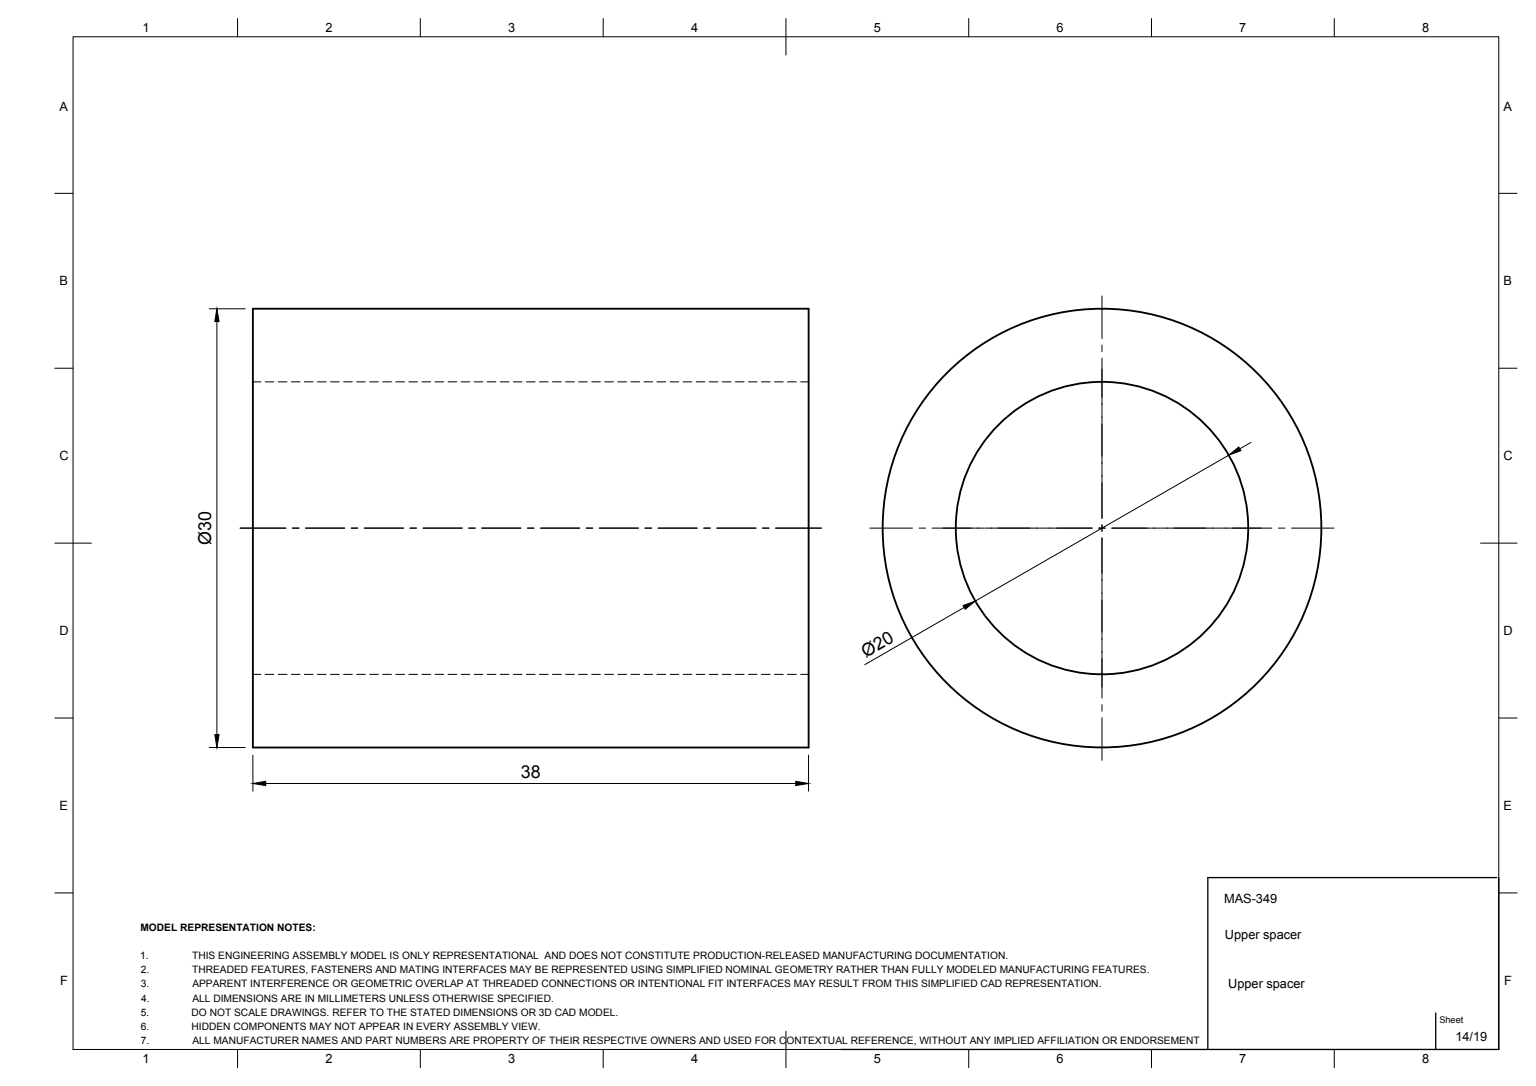
ISO-10303-21;
HEADER;
/* Generated by software containing ST-Developer
 * from STEP Tools, Inc. (www.steptools.com) 
 */

FILE_DESCRIPTION(
/* description */ ('Independent two-stage semi-open centrifugal-pump CAD. Shared impeller
s, open-machinable return casings, removable diaphragms, bronze wear/j
ournal rings, volume-preserving seal instances, retained keyed shaft, 
opposed mechanical face rings and partly threaded tie hardware. Native
 shaft rotation. Geometric topology/clearance only; flow/head/efficien
cy, pressure, cavitation, balance, preload, face loading and secondary
 seal fits/bonds, material/thermal/tolerance selection and life unassi
gned. External drive, coupling, anchors and piping bolts omitted.'),
/* implementation_level */ '2;1');

FILE_NAME(
/* name */ 'Upper spacer.step',
/* time_stamp */ '2026-11-08T18:06:32-08:00',
/* author */ (''),
/* organization */ (''),
/* preprocessor_version */ 'ST-DEVELOPER v20.2',
/* originating_system */ 'Autodesk Translation Framework v15.17.0.0',
/* authorisation */ '');

FILE_SCHEMA (('AUTOMOTIVE_DESIGN { 1 0 10303 214 3 1 1 }'));
ENDSEC;

DATA;
#10=MECHANICAL_DESIGN_GEOMETRIC_PRESENTATION_REPRESENTATION('',(#403),#16687);
#365=SHAPE_REPRESENTATION_RELATIONSHIP('SRR','None',#16774,#384);
#384=ADVANCED_BREP_SHAPE_REPRESENTATION('',(#422),#16678);
#403=STYLED_ITEM('',(#16874),#422);
#422=MANIFOLD_SOLID_BREP('Body1',#6122);
#539=FACE_BOUND('',#1424,.T.);
#540=FACE_BOUND('',#1426,.T.);
#655=PLANE('',#6849);
#656=PLANE('',#6850);
#966=FACE_OUTER_BOUND('',#1421,.T.);
#967=FACE_OUTER_BOUND('',#1422,.T.);
#968=FACE_OUTER_BOUND('',#1423,.T.);
#969=FACE_OUTER_BOUND('',#1425,.T.);
#1421=EDGE_LOOP('',(#5281,#5282,#5283,#5284));
#1422=EDGE_LOOP('',(#5285,#5286,#5287,#5288));
#1423=EDGE_LOOP('',(#5289));
#1424=EDGE_LOOP('',(#5290));
#1425=EDGE_LOOP('',(#5291));
#1426=EDGE_LOOP('',(#5292));
#1808=LINE('',#15135,#2177);
#1809=LINE('',#15141,#2178);
#2177=VECTOR('',#8302,1.);
#2178=VECTOR('',#8309,1.5);
#2458=CIRCLE('',#6844,1.);
#2459=CIRCLE('',#6845,1.);
#2460=CIRCLE('',#6847,1.5);
#2461=CIRCLE('',#6848,1.5);
#2961=VERTEX_POINT('',#15132);
#2962=VERTEX_POINT('',#15134);
#2963=VERTEX_POINT('',#15138);
#2964=VERTEX_POINT('',#15140);
#3750=EDGE_CURVE('',#2961,#2961,#2458,.T.);
#3751=EDGE_CURVE('',#2961,#2962,#1808,.T.);
#3752=EDGE_CURVE('',#2962,#2962,#2459,.T.);
#3753=EDGE_CURVE('',#2963,#2963,#2460,.T.);
#3754=EDGE_CURVE('',#2963,#2964,#1809,.T.);
#3755=EDGE_CURVE('',#2964,#2964,#2461,.T.);
#5281=ORIENTED_EDGE('',*,*,#3750,.F.);
#5282=ORIENTED_EDGE('',*,*,#3751,.T.);
#5283=ORIENTED_EDGE('',*,*,#3752,.T.);
#5284=ORIENTED_EDGE('',*,*,#3751,.F.);
#5285=ORIENTED_EDGE('',*,*,#3753,.F.);
#5286=ORIENTED_EDGE('',*,*,#3754,.T.);
#5287=ORIENTED_EDGE('',*,*,#3755,.T.);
#5288=ORIENTED_EDGE('',*,*,#3754,.F.);
#5289=ORIENTED_EDGE('',*,*,#3753,.T.);
#5290=ORIENTED_EDGE('',*,*,#3750,.T.);
#5291=ORIENTED_EDGE('',*,*,#3755,.F.);
#5292=ORIENTED_EDGE('',*,*,#3752,.F.);
#5732=CYLINDRICAL_SURFACE('',#6843,1.);
#5733=CYLINDRICAL_SURFACE('',#6846,1.5);
#6045=ADVANCED_FACE('',(#966),#5732,.F.);
#6046=ADVANCED_FACE('',(#967),#5733,.T.);
#6047=ADVANCED_FACE('',(#968,#539),#655,.T.);
#6048=ADVANCED_FACE('',(#969,#540),#656,.F.);
#6122=CLOSED_SHELL('',(#6045,#6046,#6047,#6048));
#6842=AXIS2_PLACEMENT_3D('',#15130,#8296,#8297);
#6843=AXIS2_PLACEMENT_3D('',#15131,#8298,#8299);
#6844=AXIS2_PLACEMENT_3D('',#15133,#8300,#8301);
#6845=AXIS2_PLACEMENT_3D('',#15136,#8303,#8304);
#6846=AXIS2_PLACEMENT_3D('',#15137,#8305,#8306);
#6847=AXIS2_PLACEMENT_3D('',#15139,#8307,#8308);
#6848=AXIS2_PLACEMENT_3D('',#15142,#8310,#8311);
#6849=AXIS2_PLACEMENT_3D('',#15143,#8312,#8313);
#6850=AXIS2_PLACEMENT_3D('',#15144,#8314,#8315);
#8296=DIRECTION('axis',(0.,0.,1.));
#8297=DIRECTION('refdir',(1.,0.,0.));
#8298=DIRECTION('center_axis',(0.,0.,1.));
#8299=DIRECTION('ref_axis',(1.,0.,0.));
#8300=DIRECTION('center_axis',(0.,0.,-1.));
#8301=DIRECTION('ref_axis',(1.,0.,0.));
#8302=DIRECTION('',(0.,0.,-1.));
#8303=DIRECTION('center_axis',(0.,0.,-1.));
#8304=DIRECTION('ref_axis',(1.,0.,0.));
#8305=DIRECTION('center_axis',(0.,0.,1.));
#8306=DIRECTION('ref_axis',(1.,0.,0.));
#8307=DIRECTION('center_axis',(0.,0.,1.));
#8308=DIRECTION('ref_axis',(1.,0.,0.));
#8309=DIRECTION('',(0.,0.,-1.));
#8310=DIRECTION('center_axis',(0.,0.,1.));
#8311=DIRECTION('ref_axis',(1.,0.,0.));
#8312=DIRECTION('center_axis',(0.,0.,1.));
#8313=DIRECTION('ref_axis',(1.,0.,0.));
#8314=DIRECTION('center_axis',(0.,0.,1.));
#8315=DIRECTION('ref_axis',(1.,0.,0.));
#15130=CARTESIAN_POINT('',(0.,0.,0.));
#15131=CARTESIAN_POINT('Origin',(0.,0.,7.4));
#15132=CARTESIAN_POINT('',(-1.,-1.22464679914735E-16,11.2));
#15133=CARTESIAN_POINT('Origin',(0.,0.,11.2));
#15134=CARTESIAN_POINT('',(-1.,-1.22464679914735E-16,7.4));
#15135=CARTESIAN_POINT('',(-1.,-1.22464679914735E-16,7.4));
#15136=CARTESIAN_POINT('Origin',(0.,0.,7.4));
#15137=CARTESIAN_POINT('Origin',(0.,0.,7.4));
#15138=CARTESIAN_POINT('',(-1.5,-1.83697019872103E-16,11.2));
#15139=CARTESIAN_POINT('Origin',(0.,0.,11.2));
#15140=CARTESIAN_POINT('',(-1.5,-1.83697019872103E-16,7.4));
#15141=CARTESIAN_POINT('',(-1.5,-1.83697019872103E-16,7.4));
#15142=CARTESIAN_POINT('Origin',(0.,0.,7.4));
#15143=CARTESIAN_POINT('Origin',(0.,0.,11.2));
#15144=CARTESIAN_POINT('Origin',(0.,0.,7.4));
#16657=UNCERTAINTY_MEASURE_WITH_UNIT(LENGTH_MEASURE(0.001),#16688,
'DISTANCE_ACCURACY_VALUE',
'Maximum model space distance between geometric entities at asserted c
onnectivities');
#16666=UNCERTAINTY_MEASURE_WITH_UNIT(LENGTH_MEASURE(0.001),#16688,
'DISTANCE_ACCURACY_VALUE',
'Maximum model space distance between geometric entities at asserted c
onnectivities');
#16678=(
GEOMETRIC_REPRESENTATION_CONTEXT(3)
GLOBAL_UNCERTAINTY_ASSIGNED_CONTEXT((#16657))
GLOBAL_UNIT_ASSIGNED_CONTEXT((#16688,#16690,#16691))
REPRESENTATION_CONTEXT('','3D')
);
#16687=(
GEOMETRIC_REPRESENTATION_CONTEXT(3)
GLOBAL_UNCERTAINTY_ASSIGNED_CONTEXT((#16666))
GLOBAL_UNIT_ASSIGNED_CONTEXT((#16688,#16690,#16691))
REPRESENTATION_CONTEXT('','3D')
);
#16688=(
LENGTH_UNIT()
NAMED_UNIT(*)
SI_UNIT(.CENTI.,.METRE.)
);
#16690=(
NAMED_UNIT(*)
PLANE_ANGLE_UNIT()
SI_UNIT($,.RADIAN.)
);
#16691=(
NAMED_UNIT(*)
SI_UNIT($,.STERADIAN.)
SOLID_ANGLE_UNIT()
);
#16703=SHAPE_DEFINITION_REPRESENTATION(#16723,#16774);
#16723=PRODUCT_DEFINITION_SHAPE('',$,#16795);
#16774=SHAPE_REPRESENTATION('',(#6842),#16678);
#16783=PRODUCT_DEFINITION_CONTEXT('part definition',#16845,'design');
#16795=PRODUCT_DEFINITION('Upper spacer','Upper spacer',#16815,#16783);
#16815=PRODUCT_DEFINITION_FORMATION('',$,#16858);
#16845=APPLICATION_CONTEXT(
'Core Data for Automotive Mechanical Design Process');
#16846=PRODUCT_CONTEXT('part definition',#16845,'mechanical');
#16858=PRODUCT('Upper spacer','Upper spacer',$,(#16846));
#16874=PRESENTATION_STYLE_ASSIGNMENT((#16889));
#16889=SURFACE_STYLE_USAGE(.BOTH.,#16904);
#16904=SURFACE_SIDE_STYLE('',(#16919));
#16919=SURFACE_STYLE_FILL_AREA(#16934);
#16934=FILL_AREA_STYLE('Spacer gray',(#16949));
#16949=FILL_AREA_STYLE_COLOUR('Spacer gray',#16964);
#16964=COLOUR_RGB('Spacer gray',0.576470588235294,0.615686274509804,0.666666666666667);
ENDSEC;
END-ISO-10303-21;
